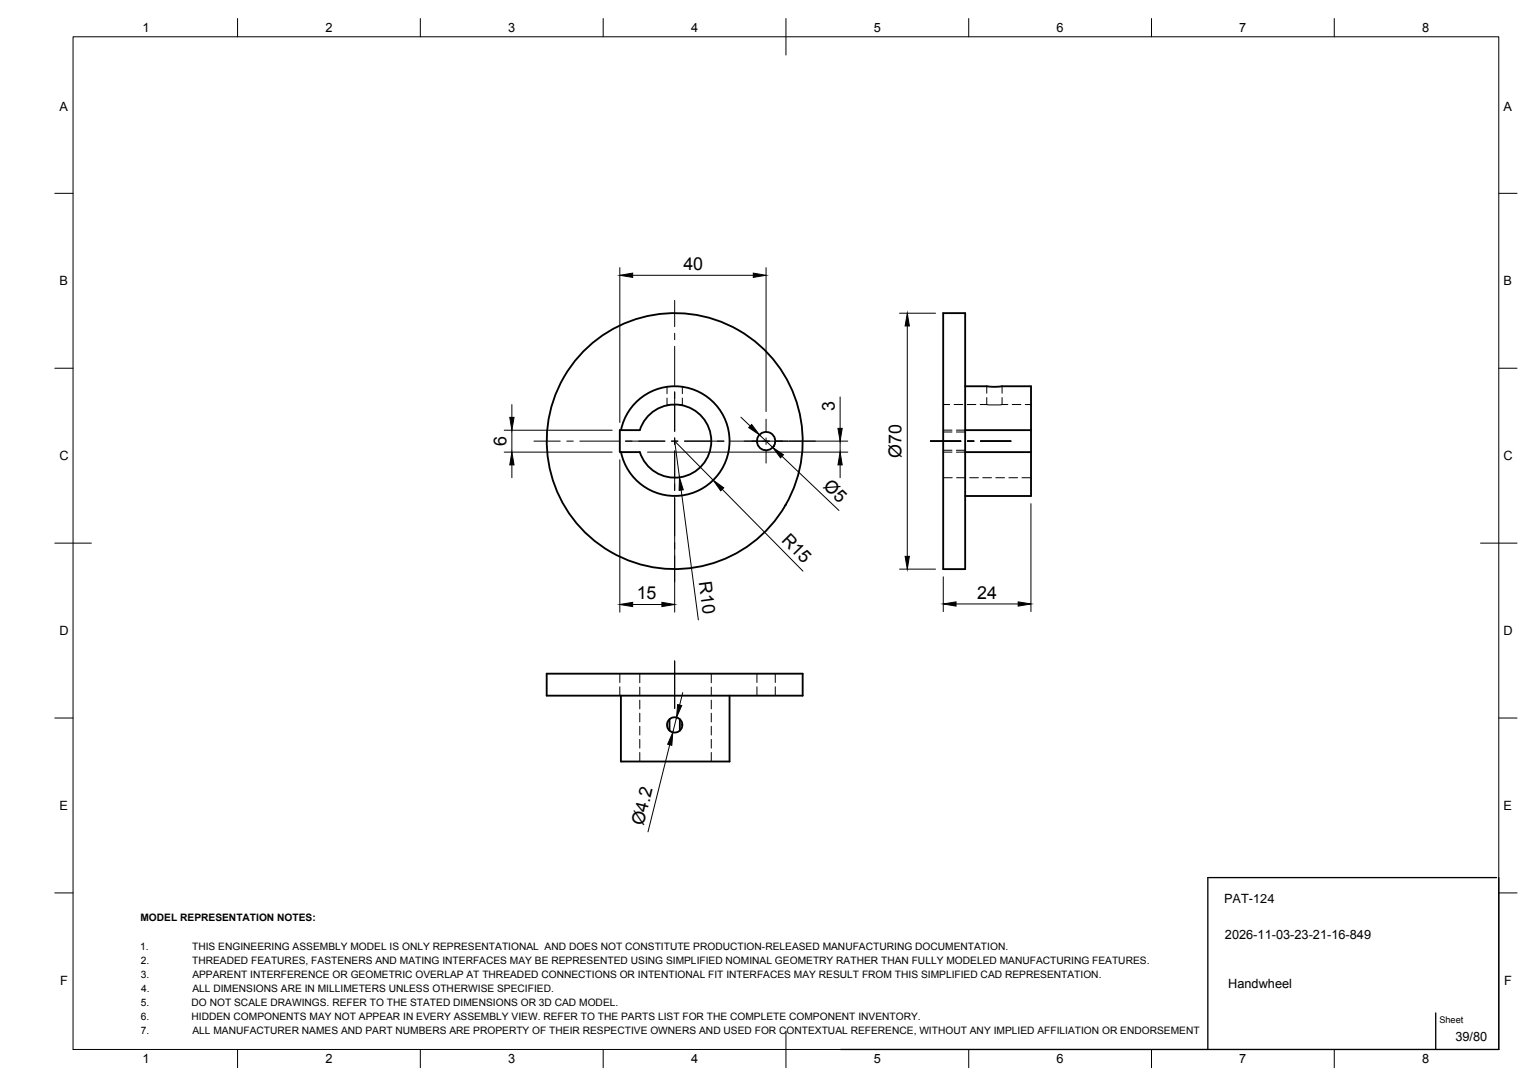
ISO-10303-21;
HEADER;
/* Generated by software containing ST-Developer
 * from STEP Tools, Inc. (www.steptools.com) 
 */

FILE_DESCRIPTION(
/* description */ ('XY cross-slide table'),
/* implementation_level */ '2;1');

FILE_NAME(
/* name */ 'Handwheel.step',
/* time_stamp */ '2026-10-28T03:22:46-07:00',
/* author */ (''),
/* organization */ (''),
/* preprocessor_version */ 'ST-DEVELOPER v20.2',
/* originating_system */ 'Autodesk Translation Framework v15.17.0.0',
/* authorisation */ '');

FILE_SCHEMA (('AUTOMOTIVE_DESIGN { 1 0 10303 214 3 1 1 }'));
ENDSEC;

DATA;
#10=MECHANICAL_DESIGN_GEOMETRIC_PRESENTATION_REPRESENTATION('',(#1720),#62984);
#1032=B_SPLINE_CURVE_WITH_KNOTS('',3,(#47403,#47404,#47405,#47406,#47407,
#47408),.UNSPECIFIED.,.F.,.F.,(4,2,4),(0.803821788694078,0.872950991853625,
0.952307212900975),.UNSPECIFIED.);
#1033=B_SPLINE_CURVE_WITH_KNOTS('',3,(#47411,#47412,#47413,#47414,#47415,
#47416,#47417,#47418,#47419,#47420),.UNSPECIFIED.,.F.,.F.,(4,2,2,2,4),(0.168950313426762,
0.238079516586309,0.317435737633658,0.396791958681008,0.465921161840561),
 .UNSPECIFIED.);
#1034=B_SPLINE_CURVE_WITH_KNOTS('',3,(#47421,#47422,#47423,#47424,#47425,
#47426),.UNSPECIFIED.,.F.,.F.,(4,2,4),(0.952307212900975,1.03166343394832,
1.10079263710787),.UNSPECIFIED.);
#1035=B_SPLINE_CURVE_WITH_KNOTS('',3,(#47430,#47431,#47432,#47433,#47434,
#47435,#47436,#47437,#47438,#47439),.UNSPECIFIED.,.F.,.F.,(4,2,2,2,4),(0.,
0.0792165807733642,0.158433161546728,0.237648697074572,0.316864232602417),
 .UNSPECIFIED.);
#1036=B_SPLINE_CURVE_WITH_KNOTS('',3,(#47440,#47441,#47442,#47443,#47444,
#47445,#47446,#47447,#47448,#47449,#47450,#47451,#47452,#47453,#47454,#47455,
#47456,#47457,#47458,#47459,#47460,#47461,#47462,#47463,#47464,#47465),
 .UNSPECIFIED.,.F.,.F.,(4,2,2,2,2,2,2,2,2,2,2,2,4),(0.316864232602417,0.396079768130261,
0.475295303658105,0.554511884431469,0.633728465204833,0.712945045978197,
0.792161626751562,0.871377162279406,0.95059269780725,1.02980823333509,1.10902376886294,
1.1882403496363,1.26745693040967),.UNSPECIFIED.);
#1539=SHAPE_REPRESENTATION_RELATIONSHIP('SRR','None',#63392,#1622);
#1622=ADVANCED_BREP_SHAPE_REPRESENTATION('',(#1830),#62929);
#1720=STYLED_ITEM('',(#63905),#1830);
#1830=MANIFOLD_SOLID_BREP('Body1',#23017);
#2071=FACE_BOUND('',#4954,.T.);
#2072=FACE_BOUND('',#4955,.T.);
#2073=FACE_BOUND('',#4957,.T.);
#2074=FACE_BOUND('',#4958,.T.);
#2075=FACE_BOUND('',#4961,.T.);
#2076=FACE_BOUND('',#4963,.T.);
#2533=PLANE('',#25052);
#2534=PLANE('',#25056);
#2535=PLANE('',#25057);
#2536=PLANE('',#25058);
#2537=PLANE('',#25059);
#2538=PLANE('',#25060);
#2539=PLANE('',#25063);
#2540=PLANE('',#25071);
#3448=FACE_OUTER_BOUND('',#4946,.T.);
#3449=FACE_OUTER_BOUND('',#4947,.T.);
#3450=FACE_OUTER_BOUND('',#4948,.T.);
#3451=FACE_OUTER_BOUND('',#4949,.T.);
#3452=FACE_OUTER_BOUND('',#4950,.T.);
#3453=FACE_OUTER_BOUND('',#4951,.T.);
#3454=FACE_OUTER_BOUND('',#4952,.T.);
#3455=FACE_OUTER_BOUND('',#4953,.T.);
#3456=FACE_OUTER_BOUND('',#4956,.T.);
#3457=FACE_OUTER_BOUND('',#4959,.T.);
#3458=FACE_OUTER_BOUND('',#4960,.T.);
#3459=FACE_OUTER_BOUND('',#4962,.T.);
#3460=FACE_OUTER_BOUND('',#4964,.T.);
#4946=EDGE_LOOP('',(#17664,#17665,#17666,#17667));
#4947=EDGE_LOOP('',(#17668,#17669));
#4948=EDGE_LOOP('',(#17670,#17671,#17672,#17673,#17674,#17675,#17676,#17677,
#17678));
#4949=EDGE_LOOP('',(#17679,#17680));
#4950=EDGE_LOOP('',(#17681,#17682,#17683,#17684,#17685,#17686));
#4951=EDGE_LOOP('',(#17687,#17688,#17689,#17690));
#4952=EDGE_LOOP('',(#17691,#17692,#17693,#17694,#17695,#17696));
#4953=EDGE_LOOP('',(#17697));
#4954=EDGE_LOOP('',(#17698));
#4955=EDGE_LOOP('',(#17699,#17700,#17701,#17702));
#4956=EDGE_LOOP('',(#17703));
#4957=EDGE_LOOP('',(#17704));
#4958=EDGE_LOOP('',(#17705,#17706,#17707,#17708));
#4959=EDGE_LOOP('',(#17709,#17710,#17711,#17712));
#4960=EDGE_LOOP('',(#17713,#17714,#17715,#17716));
#4961=EDGE_LOOP('',(#17717,#17718,#17719,#17720,#17721));
#4962=EDGE_LOOP('',(#17722,#17723,#17724,#17725));
#4963=EDGE_LOOP('',(#17726,#17727));
#4964=EDGE_LOOP('',(#17728,#17729,#17730,#17731));
#6550=LINE('',#47393,#8037);
#6551=LINE('',#47398,#8038);
#6552=LINE('',#47428,#8039);
#6553=LINE('',#47467,#8040);
#6554=LINE('',#47471,#8041);
#6555=LINE('',#47473,#8042);
#6556=LINE('',#47475,#8043);
#6557=LINE('',#47477,#8044);
#6558=LINE('',#47479,#8045);
#6559=LINE('',#47480,#8046);
#6560=LINE('',#47483,#8047);
#6561=LINE('',#47485,#8048);
#6562=LINE('',#47486,#8049);
#6563=LINE('',#47489,#8050);
#6564=LINE('',#47491,#8051);
#6565=LINE('',#47493,#8052);
#6566=LINE('',#47495,#8053);
#6567=LINE('',#47496,#8054);
#6568=LINE('',#47506,#8055);
#8037=VECTOR('',#29207,0.25);
#8038=VECTOR('',#29212,1.);
#8039=VECTOR('',#29219,0.210000000000001);
#8040=VECTOR('',#29222,1.);
#8041=VECTOR('',#29225,1.);
#8042=VECTOR('',#29226,1.);
#8043=VECTOR('',#29227,1.);
#8044=VECTOR('',#29228,1.);
#8045=VECTOR('',#29229,1.);
#8046=VECTOR('',#29230,1.);
#8047=VECTOR('',#29233,1.);
#8048=VECTOR('',#29234,1.);
#8049=VECTOR('',#29235,1.);
#8050=VECTOR('',#29238,1.);
#8051=VECTOR('',#29239,1.);
#8052=VECTOR('',#29240,1.);
#8053=VECTOR('',#29241,1.);
#8054=VECTOR('',#29242,1.);
#8055=VECTOR('',#29257,3.5);
#9277=CIRCLE('',#25050,0.25);
#9278=CIRCLE('',#25051,0.25);
#9279=CIRCLE('',#25053,0.210000000000001);
#9280=CIRCLE('',#25055,0.210000000000001);
#9281=CIRCLE('',#25061,3.5);
#9282=CIRCLE('',#25062,1.);
#9283=CIRCLE('',#25064,3.5);
#9284=CIRCLE('',#25065,1.5);
#9285=CIRCLE('',#25068,1.);
#9286=CIRCLE('',#25070,1.5);
#10704=VERTEX_POINT('',#47390);
#10705=VERTEX_POINT('',#47392);
#10706=VERTEX_POINT('',#47396);
#10707=VERTEX_POINT('',#47397);
#10708=VERTEX_POINT('',#47401);
#10709=VERTEX_POINT('',#47402);
#10710=VERTEX_POINT('',#47409);
#10711=VERTEX_POINT('',#47427);
#10712=VERTEX_POINT('',#47429);
#10713=VERTEX_POINT('',#47469);
#10714=VERTEX_POINT('',#47470);
#10715=VERTEX_POINT('',#47472);
#10716=VERTEX_POINT('',#47474);
#10717=VERTEX_POINT('',#47476);
#10718=VERTEX_POINT('',#47478);
#10719=VERTEX_POINT('',#47482);
#10720=VERTEX_POINT('',#47484);
#10721=VERTEX_POINT('',#47488);
#10722=VERTEX_POINT('',#47490);
#10723=VERTEX_POINT('',#47492);
#10724=VERTEX_POINT('',#47494);
#10725=VERTEX_POINT('',#47498);
#10726=VERTEX_POINT('',#47502);
#13216=EDGE_CURVE('',#10704,#10704,#9277,.T.);
#13217=EDGE_CURVE('',#10704,#10705,#6550,.T.);
#13218=EDGE_CURVE('',#10705,#10705,#9278,.T.);
#13219=EDGE_CURVE('',#10706,#10707,#6551,.T.);
#13220=EDGE_CURVE('',#10706,#10707,#9279,.T.);
#13221=EDGE_CURVE('',#10708,#10709,#1032,.T.);
#13222=EDGE_CURVE('',#10710,#10708,#9280,.T.);
#13223=EDGE_CURVE('',#10707,#10710,#1033,.T.);
#13224=EDGE_CURVE('',#10709,#10706,#1034,.T.);
#13225=EDGE_CURVE('',#10709,#10711,#6552,.T.);
#13226=EDGE_CURVE('',#10712,#10711,#1035,.T.);
#13227=EDGE_CURVE('',#10711,#10712,#1036,.T.);
#13228=EDGE_CURVE('',#10710,#10708,#6553,.T.);
#13229=EDGE_CURVE('',#10713,#10714,#6554,.T.);
#13230=EDGE_CURVE('',#10715,#10713,#6555,.T.);
#13231=EDGE_CURVE('',#10716,#10715,#6556,.T.);
#13232=EDGE_CURVE('',#10717,#10716,#6557,.T.);
#13233=EDGE_CURVE('',#10718,#10717,#6558,.T.);
#13234=EDGE_CURVE('',#10714,#10718,#6559,.T.);
#13235=EDGE_CURVE('',#10719,#10713,#6560,.T.);
#13236=EDGE_CURVE('',#10720,#10719,#6561,.T.);
#13237=EDGE_CURVE('',#10715,#10720,#6562,.T.);
#13238=EDGE_CURVE('',#10721,#10719,#6563,.T.);
#13239=EDGE_CURVE('',#10722,#10721,#6564,.T.);
#13240=EDGE_CURVE('',#10723,#10722,#6565,.T.);
#13241=EDGE_CURVE('',#10724,#10723,#6566,.T.);
#13242=EDGE_CURVE('',#10720,#10724,#6567,.T.);
#13243=EDGE_CURVE('',#10725,#10725,#9281,.T.);
#13244=EDGE_CURVE('',#10714,#10721,#9282,.T.);
#13245=EDGE_CURVE('',#10726,#10726,#9283,.T.);
#13246=EDGE_CURVE('',#10724,#10716,#9284,.T.);
#13247=EDGE_CURVE('',#10725,#10726,#6568,.T.);
#13248=EDGE_CURVE('',#10718,#10722,#9285,.T.);
#13249=EDGE_CURVE('',#10723,#10717,#9286,.T.);
#17664=ORIENTED_EDGE('',*,*,#13216,.F.);
#17665=ORIENTED_EDGE('',*,*,#13217,.T.);
#17666=ORIENTED_EDGE('',*,*,#13218,.F.);
#17667=ORIENTED_EDGE('',*,*,#13217,.F.);
#17668=ORIENTED_EDGE('',*,*,#13219,.F.);
#17669=ORIENTED_EDGE('',*,*,#13220,.T.);
#17670=ORIENTED_EDGE('',*,*,#13221,.F.);
#17671=ORIENTED_EDGE('',*,*,#13222,.F.);
#17672=ORIENTED_EDGE('',*,*,#13223,.F.);
#17673=ORIENTED_EDGE('',*,*,#13220,.F.);
#17674=ORIENTED_EDGE('',*,*,#13224,.F.);
#17675=ORIENTED_EDGE('',*,*,#13225,.T.);
#17676=ORIENTED_EDGE('',*,*,#13226,.F.);
#17677=ORIENTED_EDGE('',*,*,#13227,.F.);
#17678=ORIENTED_EDGE('',*,*,#13225,.F.);
#17679=ORIENTED_EDGE('',*,*,#13228,.F.);
#17680=ORIENTED_EDGE('',*,*,#13222,.T.);
#17681=ORIENTED_EDGE('',*,*,#13229,.F.);
#17682=ORIENTED_EDGE('',*,*,#13230,.F.);
#17683=ORIENTED_EDGE('',*,*,#13231,.F.);
#17684=ORIENTED_EDGE('',*,*,#13232,.F.);
#17685=ORIENTED_EDGE('',*,*,#13233,.F.);
#17686=ORIENTED_EDGE('',*,*,#13234,.F.);
#17687=ORIENTED_EDGE('',*,*,#13235,.F.);
#17688=ORIENTED_EDGE('',*,*,#13236,.F.);
#17689=ORIENTED_EDGE('',*,*,#13237,.F.);
#17690=ORIENTED_EDGE('',*,*,#13230,.T.);
#17691=ORIENTED_EDGE('',*,*,#13238,.F.);
#17692=ORIENTED_EDGE('',*,*,#13239,.F.);
#17693=ORIENTED_EDGE('',*,*,#13240,.F.);
#17694=ORIENTED_EDGE('',*,*,#13241,.F.);
#17695=ORIENTED_EDGE('',*,*,#13242,.F.);
#17696=ORIENTED_EDGE('',*,*,#13236,.T.);
#17697=ORIENTED_EDGE('',*,*,#13243,.T.);
#17698=ORIENTED_EDGE('',*,*,#13218,.T.);
#17699=ORIENTED_EDGE('',*,*,#13238,.T.);
#17700=ORIENTED_EDGE('',*,*,#13235,.T.);
#17701=ORIENTED_EDGE('',*,*,#13229,.T.);
#17702=ORIENTED_EDGE('',*,*,#13244,.T.);
#17703=ORIENTED_EDGE('',*,*,#13245,.F.);
#17704=ORIENTED_EDGE('',*,*,#13216,.T.);
#17705=ORIENTED_EDGE('',*,*,#13242,.T.);
#17706=ORIENTED_EDGE('',*,*,#13246,.T.);
#17707=ORIENTED_EDGE('',*,*,#13231,.T.);
#17708=ORIENTED_EDGE('',*,*,#13237,.T.);
#17709=ORIENTED_EDGE('',*,*,#13243,.F.);
#17710=ORIENTED_EDGE('',*,*,#13247,.T.);
#17711=ORIENTED_EDGE('',*,*,#13245,.T.);
#17712=ORIENTED_EDGE('',*,*,#13247,.F.);
#17713=ORIENTED_EDGE('',*,*,#13239,.T.);
#17714=ORIENTED_EDGE('',*,*,#13244,.F.);
#17715=ORIENTED_EDGE('',*,*,#13234,.T.);
#17716=ORIENTED_EDGE('',*,*,#13248,.T.);
#17717=ORIENTED_EDGE('',*,*,#13223,.T.);
#17718=ORIENTED_EDGE('',*,*,#13228,.T.);
#17719=ORIENTED_EDGE('',*,*,#13221,.T.);
#17720=ORIENTED_EDGE('',*,*,#13224,.T.);
#17721=ORIENTED_EDGE('',*,*,#13219,.T.);
#17722=ORIENTED_EDGE('',*,*,#13241,.T.);
#17723=ORIENTED_EDGE('',*,*,#13249,.T.);
#17724=ORIENTED_EDGE('',*,*,#13232,.T.);
#17725=ORIENTED_EDGE('',*,*,#13246,.F.);
#17726=ORIENTED_EDGE('',*,*,#13226,.T.);
#17727=ORIENTED_EDGE('',*,*,#13227,.T.);
#17728=ORIENTED_EDGE('',*,*,#13240,.T.);
#17729=ORIENTED_EDGE('',*,*,#13248,.F.);
#17730=ORIENTED_EDGE('',*,*,#13233,.T.);
#17731=ORIENTED_EDGE('',*,*,#13249,.F.);
#21324=CYLINDRICAL_SURFACE('',#25049,0.25);
#21325=CYLINDRICAL_SURFACE('',#25054,0.210000000000001);
#21326=CYLINDRICAL_SURFACE('',#25066,3.5);
#21327=CYLINDRICAL_SURFACE('',#25067,1.);
#21328=CYLINDRICAL_SURFACE('',#25069,1.5);
#22229=ADVANCED_FACE('',(#3448),#21324,.F.);
#22230=ADVANCED_FACE('',(#3449),#2533,.T.);
#22231=ADVANCED_FACE('',(#3450),#21325,.F.);
#22232=ADVANCED_FACE('',(#3451),#2534,.T.);
#22233=ADVANCED_FACE('',(#3452),#2535,.F.);
#22234=ADVANCED_FACE('',(#3453),#2536,.F.);
#22235=ADVANCED_FACE('',(#3454),#2537,.F.);
#22236=ADVANCED_FACE('',(#3455,#2071,#2072),#2538,.T.);
#22237=ADVANCED_FACE('',(#3456,#2073,#2074),#2539,.F.);
#22238=ADVANCED_FACE('',(#3457),#21326,.T.);
#22239=ADVANCED_FACE('',(#3458,#2075),#21327,.F.);
#22240=ADVANCED_FACE('',(#3459,#2076),#21328,.T.);
#22241=ADVANCED_FACE('',(#3460),#2540,.F.);
#23017=CLOSED_SHELL('',(#22229,#22230,#22231,#22232,#22233,#22234,#22235,
#22236,#22237,#22238,#22239,#22240,#22241));
#25048=AXIS2_PLACEMENT_3D('',#47388,#29201,#29202);
#25049=AXIS2_PLACEMENT_3D('',#47389,#29203,#29204);
#25050=AXIS2_PLACEMENT_3D('',#47391,#29205,#29206);
#25051=AXIS2_PLACEMENT_3D('',#47394,#29208,#29209);
#25052=AXIS2_PLACEMENT_3D('',#47395,#29210,#29211);
#25053=AXIS2_PLACEMENT_3D('',#47399,#29213,#29214);
#25054=AXIS2_PLACEMENT_3D('',#47400,#29215,#29216);
#25055=AXIS2_PLACEMENT_3D('',#47410,#29217,#29218);
#25056=AXIS2_PLACEMENT_3D('',#47466,#29220,#29221);
#25057=AXIS2_PLACEMENT_3D('',#47468,#29223,#29224);
#25058=AXIS2_PLACEMENT_3D('',#47481,#29231,#29232);
#25059=AXIS2_PLACEMENT_3D('',#47487,#29236,#29237);
#25060=AXIS2_PLACEMENT_3D('',#47497,#29243,#29244);
#25061=AXIS2_PLACEMENT_3D('',#47499,#29245,#29246);
#25062=AXIS2_PLACEMENT_3D('',#47500,#29247,#29248);
#25063=AXIS2_PLACEMENT_3D('',#47501,#29249,#29250);
#25064=AXIS2_PLACEMENT_3D('',#47503,#29251,#29252);
#25065=AXIS2_PLACEMENT_3D('',#47504,#29253,#29254);
#25066=AXIS2_PLACEMENT_3D('',#47505,#29255,#29256);
#25067=AXIS2_PLACEMENT_3D('',#47507,#29258,#29259);
#25068=AXIS2_PLACEMENT_3D('',#47508,#29260,#29261);
#25069=AXIS2_PLACEMENT_3D('',#47509,#29262,#29263);
#25070=AXIS2_PLACEMENT_3D('',#47510,#29264,#29265);
#25071=AXIS2_PLACEMENT_3D('',#47511,#29266,#29267);
#29201=DIRECTION('axis',(0.,0.,1.));
#29202=DIRECTION('refdir',(1.,0.,0.));
#29203=DIRECTION('center_axis',(1.,0.,0.));
#29204=DIRECTION('ref_axis',(0.,0.,-1.));
#29205=DIRECTION('center_axis',(1.,0.,0.));
#29206=DIRECTION('ref_axis',(0.,0.,-1.));
#29207=DIRECTION('',(1.,0.,0.));
#29208=DIRECTION('center_axis',(-1.,0.,0.));
#29209=DIRECTION('ref_axis',(0.,0.,-1.));
#29210=DIRECTION('center_axis',(0.,1.,0.));
#29211=DIRECTION('ref_axis',(1.,0.,0.));
#29212=DIRECTION('',(1.,0.,0.));
#29213=DIRECTION('center_axis',(0.,1.,0.));
#29214=DIRECTION('ref_axis',(1.,0.,0.));
#29215=DIRECTION('center_axis',(0.,1.,0.));
#29216=DIRECTION('ref_axis',(1.,0.,0.));
#29217=DIRECTION('center_axis',(0.,1.,0.));
#29218=DIRECTION('ref_axis',(1.,0.,0.));
#29219=DIRECTION('',(0.,1.,0.));
#29220=DIRECTION('center_axis',(0.,1.,0.));
#29221=DIRECTION('ref_axis',(1.,0.,0.));
#29222=DIRECTION('',(-1.,0.,0.));
#29223=DIRECTION('center_axis',(0.,-1.,0.));
#29224=DIRECTION('ref_axis',(0.,0.,-1.));
#29225=DIRECTION('',(0.,0.,1.));
#29226=DIRECTION('',(1.,0.,0.));
#29227=DIRECTION('',(0.,0.,-1.));
#29228=DIRECTION('',(1.,0.,0.));
#29229=DIRECTION('',(0.,0.,-1.));
#29230=DIRECTION('',(-1.,0.,0.));
#29231=DIRECTION('center_axis',(0.,0.,-1.));
#29232=DIRECTION('ref_axis',(0.,1.,0.));
#29233=DIRECTION('',(0.,-1.,0.));
#29234=DIRECTION('',(1.,0.,0.));
#29235=DIRECTION('',(0.,1.,0.));
#29236=DIRECTION('center_axis',(0.,1.,0.));
#29237=DIRECTION('ref_axis',(0.,0.,1.));
#29238=DIRECTION('',(0.,0.,-1.));
#29239=DIRECTION('',(1.,0.,0.));
#29240=DIRECTION('',(0.,0.,1.));
#29241=DIRECTION('',(-1.,0.,0.));
#29242=DIRECTION('',(0.,0.,1.));
#29243=DIRECTION('center_axis',(1.,0.,0.));
#29244=DIRECTION('ref_axis',(0.,0.,-1.));
#29245=DIRECTION('center_axis',(1.,0.,0.));
#29246=DIRECTION('ref_axis',(0.,0.,-1.));
#29247=DIRECTION('center_axis',(-1.,0.,0.));
#29248=DIRECTION('ref_axis',(0.,0.,-1.));
#29249=DIRECTION('center_axis',(1.,0.,0.));
#29250=DIRECTION('ref_axis',(0.,0.,-1.));
#29251=DIRECTION('center_axis',(1.,0.,0.));
#29252=DIRECTION('ref_axis',(0.,0.,-1.));
#29253=DIRECTION('center_axis',(1.,0.,0.));
#29254=DIRECTION('ref_axis',(0.,0.,-1.));
#29255=DIRECTION('center_axis',(1.,0.,0.));
#29256=DIRECTION('ref_axis',(0.,0.,-1.));
#29257=DIRECTION('',(-1.,0.,0.));
#29258=DIRECTION('center_axis',(1.,0.,0.));
#29259=DIRECTION('ref_axis',(0.,1.22464679914735E-16,1.));
#29260=DIRECTION('center_axis',(-1.,0.,0.));
#29261=DIRECTION('ref_axis',(0.,0.,-1.));
#29262=DIRECTION('center_axis',(1.,0.,0.));
#29263=DIRECTION('ref_axis',(0.,1.22464679914735E-16,1.));
#29264=DIRECTION('center_axis',(1.,0.,0.));
#29265=DIRECTION('ref_axis',(0.,0.,-1.));
#29266=DIRECTION('center_axis',(1.,0.,0.));
#29267=DIRECTION('ref_axis',(0.,0.,-1.));
#47388=CARTESIAN_POINT('',(0.,0.,0.));
#47389=CARTESIAN_POINT('Origin',(28.7,0.,6.5));
#47390=CARTESIAN_POINT('',(28.8,-3.06161699786838E-17,6.75));
#47391=CARTESIAN_POINT('Origin',(28.8,0.,6.5));
#47392=CARTESIAN_POINT('',(29.4,3.06161699786838E-17,6.75));
#47393=CARTESIAN_POINT('',(28.7,-3.06161699786838E-17,6.75));
#47394=CARTESIAN_POINT('Origin',(29.4,0.,6.5));
#47395=CARTESIAN_POINT('Origin',(28.,0.99,4.));
#47396=CARTESIAN_POINT('',(27.844436508139,0.99,4.14106735979666));
#47397=CARTESIAN_POINT('',(28.155563491861,0.99,4.14106735979666));
#47398=CARTESIAN_POINT('',(27.,0.99,4.14106735979666));
#47399=CARTESIAN_POINT('Origin',(28.,0.99,4.));
#47400=CARTESIAN_POINT('Origin',(28.,0.99,4.));
#47401=CARTESIAN_POINT('',(27.844436508139,0.99,3.85893264020334));
#47402=CARTESIAN_POINT('',(27.79,1.,4.));
#47403=CARTESIAN_POINT('Ctrl Pts',(27.844436508139,0.99,3.85893264020334));
#47404=CARTESIAN_POINT('Ctrl Pts',(27.8287948476368,0.992457849824465,3.87618164330178));
#47405=CARTESIAN_POINT('Ctrl Pts',(27.815375956669,0.994938193049464,3.8970013568903));
#47406=CARTESIAN_POINT('Ctrl Pts',(27.7953025362756,0.998844492372413,3.94538588560165));
#47407=CARTESIAN_POINT('Ctrl Pts',(27.79,1.,3.97354792631755));
#47408=CARTESIAN_POINT('Ctrl Pts',(27.79,1.,4.));
#47409=CARTESIAN_POINT('',(28.155563491861,0.99,3.85893264020334));
#47410=CARTESIAN_POINT('Origin',(28.,0.99,4.));
#47411=CARTESIAN_POINT('Ctrl Pts',(28.155563491861,0.99,4.14106735979666));
#47412=CARTESIAN_POINT('Ctrl Pts',(28.1712051523632,0.992457849824465,4.12381835669823));
#47413=CARTESIAN_POINT('Ctrl Pts',(28.184624043331,0.994938193049464,4.1029986431097));
#47414=CARTESIAN_POINT('Ctrl Pts',(28.2046974637244,0.998844492372413,4.05461411439835));
#47415=CARTESIAN_POINT('Ctrl Pts',(28.21,1.,4.02645207368245));
#47416=CARTESIAN_POINT('Ctrl Pts',(28.21,1.,3.97354792631755));
#47417=CARTESIAN_POINT('Ctrl Pts',(28.2046974637244,0.998844492372413,3.94538588560165));
#47418=CARTESIAN_POINT('Ctrl Pts',(28.184624043331,0.994938193049464,3.8970013568903));
#47419=CARTESIAN_POINT('Ctrl Pts',(28.1712051523632,0.992457849824465,3.87618164330178));
#47420=CARTESIAN_POINT('Ctrl Pts',(28.155563491861,0.99,3.85893264020334));
#47421=CARTESIAN_POINT('Ctrl Pts',(27.79,1.,4.));
#47422=CARTESIAN_POINT('Ctrl Pts',(27.79,1.,4.02645207368245));
#47423=CARTESIAN_POINT('Ctrl Pts',(27.7953025362756,0.998844492372413,4.05461411439835));
#47424=CARTESIAN_POINT('Ctrl Pts',(27.815375956669,0.994938193049464,4.1029986431097));
#47425=CARTESIAN_POINT('Ctrl Pts',(27.8287948476368,0.992457849824465,4.12381835669823));
#47426=CARTESIAN_POINT('Ctrl Pts',(27.844436508139,0.99,4.14106735979666));
#47427=CARTESIAN_POINT('',(27.79,1.5,4.));
#47428=CARTESIAN_POINT('',(27.79,0.99,4.));
#47429=CARTESIAN_POINT('',(28.,1.48522725533839,4.21));
#47430=CARTESIAN_POINT('Ctrl Pts',(28.,1.48522725533839,4.21));
#47431=CARTESIAN_POINT('Ctrl Pts',(27.9735944730755,1.48522725533839,4.21));
#47432=CARTESIAN_POINT('Ctrl Pts',(27.9454529259093,1.48600415954412,4.20471573726959));
#47433=CARTESIAN_POINT('Ctrl Pts',(27.8937237310949,1.48880073282317,4.18327376303633));
#47434=CARTESIAN_POINT('Ctrl Pts',(27.870133075872,1.49077897157582,4.16711792397039));
#47435=CARTESIAN_POINT('Ctrl Pts',(27.832882321789,1.49448481141327,4.12986716988737));
#47436=CARTESIAN_POINT('Ctrl Pts',(27.8167262899986,1.49645455657129,4.10627640830576));
#47437=CARTESIAN_POINT('Ctrl Pts',(27.7952841751738,1.49923165515646,4.0545468514059));
#47438=CARTESIAN_POINT('Ctrl Pts',(27.79,1.5,4.02640517850928));
#47439=CARTESIAN_POINT('Ctrl Pts',(27.79,1.5,4.));
#47440=CARTESIAN_POINT('Ctrl Pts',(27.79,1.5,4.));
#47441=CARTESIAN_POINT('Ctrl Pts',(27.79,1.5,3.97359482149072));
#47442=CARTESIAN_POINT('Ctrl Pts',(27.7952841751738,1.49923165515646,3.9454531485941));
#47443=CARTESIAN_POINT('Ctrl Pts',(27.8167262899986,1.49645455657129,3.89372359169424));
#47444=CARTESIAN_POINT('Ctrl Pts',(27.832882321789,1.49448481141327,3.87013283011263));
#47445=CARTESIAN_POINT('Ctrl Pts',(27.870133075872,1.49077897157582,3.83288207602961));
#47446=CARTESIAN_POINT('Ctrl Pts',(27.8937237310949,1.48880073282317,3.81672623696367));
#47447=CARTESIAN_POINT('Ctrl Pts',(27.9454529259093,1.48600415954412,3.7952842627304));
#47448=CARTESIAN_POINT('Ctrl Pts',(27.9735944730755,1.48522725533839,3.79));
#47449=CARTESIAN_POINT('Ctrl Pts',(28.0264055269245,1.48522725533839,3.79));
#47450=CARTESIAN_POINT('Ctrl Pts',(28.0545470740907,1.48600415954412,3.7952842627304));
#47451=CARTESIAN_POINT('Ctrl Pts',(28.1062762689051,1.48880073282317,3.81672623696367));
#47452=CARTESIAN_POINT('Ctrl Pts',(28.129866924128,1.49077897157582,3.83288207602961));
#47453=CARTESIAN_POINT('Ctrl Pts',(28.167117678211,1.49448481141327,3.87013283011263));
#47454=CARTESIAN_POINT('Ctrl Pts',(28.1832737100014,1.49645455657129,3.89372359169424));
#47455=CARTESIAN_POINT('Ctrl Pts',(28.2047158248262,1.49923165515646,3.9454531485941));
#47456=CARTESIAN_POINT('Ctrl Pts',(28.21,1.5,3.97359482149072));
#47457=CARTESIAN_POINT('Ctrl Pts',(28.21,1.5,4.02640517850928));
#47458=CARTESIAN_POINT('Ctrl Pts',(28.2047158248262,1.49923165515646,4.0545468514059));
#47459=CARTESIAN_POINT('Ctrl Pts',(28.1832737100014,1.49645455657129,4.10627640830576));
#47460=CARTESIAN_POINT('Ctrl Pts',(28.167117678211,1.49448481141327,4.12986716988737));
#47461=CARTESIAN_POINT('Ctrl Pts',(28.129866924128,1.49077897157582,4.16711792397039));
#47462=CARTESIAN_POINT('Ctrl Pts',(28.1062762689051,1.48880073282317,4.18327376303633));
#47463=CARTESIAN_POINT('Ctrl Pts',(28.0545470740907,1.48600415954412,4.2047157372696));
#47464=CARTESIAN_POINT('Ctrl Pts',(28.0264055269245,1.48522725533839,4.21));
#47465=CARTESIAN_POINT('Ctrl Pts',(28.,1.48522725533839,4.21));
#47466=CARTESIAN_POINT('Origin',(28.,0.99,4.));
#47467=CARTESIAN_POINT('',(27.,0.99,3.85893264020334));
#47468=CARTESIAN_POINT('Origin',(26.9,-0.3,4.));
#47469=CARTESIAN_POINT('',(29.4,-0.3,2.5));
#47470=CARTESIAN_POINT('',(29.4,-0.3,3.04606079858305));
#47471=CARTESIAN_POINT('',(29.4,-0.3,4.));
#47472=CARTESIAN_POINT('',(28.8,-0.3,2.5));
#47473=CARTESIAN_POINT('',(26.9,-0.3,2.5));
#47474=CARTESIAN_POINT('',(28.8,-0.3,2.53030615433009));
#47475=CARTESIAN_POINT('',(28.8,-0.3,4.));
#47476=CARTESIAN_POINT('',(27.,-0.3,2.53030615433009));
#47477=CARTESIAN_POINT('',(27.,-0.3,2.53030615433009));
#47478=CARTESIAN_POINT('',(27.,-0.3,3.04606079858305));
#47479=CARTESIAN_POINT('',(27.,-0.3,4.));
#47480=CARTESIAN_POINT('',(27.,-0.3,3.04606079858305));
#47481=CARTESIAN_POINT('Origin',(26.9,-0.3,2.5));
#47482=CARTESIAN_POINT('',(29.4,0.3,2.5));
#47483=CARTESIAN_POINT('',(29.4,-0.15,2.5));
#47484=CARTESIAN_POINT('',(28.8,0.3,2.5));
#47485=CARTESIAN_POINT('',(26.9,0.3,2.5));
#47486=CARTESIAN_POINT('',(28.8,-0.15,2.5));
#47487=CARTESIAN_POINT('Origin',(26.9,0.3,2.5));
#47488=CARTESIAN_POINT('',(29.4,0.3,3.04606079858305));
#47489=CARTESIAN_POINT('',(29.4,0.3,3.25));
#47490=CARTESIAN_POINT('',(27.,0.3,3.04606079858305));
#47491=CARTESIAN_POINT('',(27.,0.3,3.04606079858305));
#47492=CARTESIAN_POINT('',(27.,0.3,2.53030615433009));
#47493=CARTESIAN_POINT('',(27.,0.3,3.25));
#47494=CARTESIAN_POINT('',(28.8,0.3,2.53030615433009));
#47495=CARTESIAN_POINT('',(27.,0.3,2.53030615433009));
#47496=CARTESIAN_POINT('',(28.8,0.3,3.25));
#47497=CARTESIAN_POINT('Origin',(29.4,0.,4.));
#47498=CARTESIAN_POINT('',(29.4,-4.28626379701574E-16,7.5));
#47499=CARTESIAN_POINT('Origin',(29.4,0.,4.));
#47500=CARTESIAN_POINT('Origin',(29.4,0.,4.));
#47501=CARTESIAN_POINT('Origin',(28.8,0.,4.));
#47502=CARTESIAN_POINT('',(28.8,-4.28626379701574E-16,7.5));
#47503=CARTESIAN_POINT('Origin',(28.8,0.,4.));
#47504=CARTESIAN_POINT('Origin',(28.8,0.,4.));
#47505=CARTESIAN_POINT('Origin',(28.8,0.,4.));
#47506=CARTESIAN_POINT('',(28.8,-4.28626379701574E-16,7.5));
#47507=CARTESIAN_POINT('Origin',(27.,0.,4.));
#47508=CARTESIAN_POINT('Origin',(27.,0.,4.));
#47509=CARTESIAN_POINT('Origin',(27.,0.,4.));
#47510=CARTESIAN_POINT('Origin',(27.,0.,4.));
#47511=CARTESIAN_POINT('Origin',(27.,0.,4.));
#62830=UNCERTAINTY_MEASURE_WITH_UNIT(LENGTH_MEASURE(0.001),#62985,
'DISTANCE_ACCURACY_VALUE',
'Maximum model space distance between geometric entities at asserted c
onnectivities');
#62885=UNCERTAINTY_MEASURE_WITH_UNIT(LENGTH_MEASURE(0.001),#62985,
'DISTANCE_ACCURACY_VALUE',
'Maximum model space distance between geometric entities at asserted c
onnectivities');
#62929=(
GEOMETRIC_REPRESENTATION_CONTEXT(3)
GLOBAL_UNCERTAINTY_ASSIGNED_CONTEXT((#62830))
GLOBAL_UNIT_ASSIGNED_CONTEXT((#62985,#62987,#62988))
REPRESENTATION_CONTEXT('','3D')
);
#62984=(
GEOMETRIC_REPRESENTATION_CONTEXT(3)
GLOBAL_UNCERTAINTY_ASSIGNED_CONTEXT((#62885))
GLOBAL_UNIT_ASSIGNED_CONTEXT((#62985,#62987,#62988))
REPRESENTATION_CONTEXT('','3D')
);
#62985=(
LENGTH_UNIT()
NAMED_UNIT(*)
SI_UNIT(.CENTI.,.METRE.)
);
#62987=(
NAMED_UNIT(*)
PLANE_ANGLE_UNIT()
SI_UNIT($,.RADIAN.)
);
#62988=(
NAMED_UNIT(*)
SI_UNIT($,.STERADIAN.)
SOLID_ANGLE_UNIT()
);
#63032=SHAPE_DEFINITION_REPRESENTATION(#63163,#63392);
#63163=PRODUCT_DEFINITION_SHAPE('',$,#63491);
#63392=SHAPE_REPRESENTATION('',(#25048),#62929);
#63447=PRODUCT_DEFINITION_CONTEXT('part definition',#63743,'design');
#63491=PRODUCT_DEFINITION('Handwheel','Handwheel',#63589,#63447);
#63589=PRODUCT_DEFINITION_FORMATION('',$,#63788);
#63743=APPLICATION_CONTEXT(
'Core Data for Automotive Mechanical Design Process');
#63744=PRODUCT_CONTEXT('part definition',#63743,'mechanical');
#63788=PRODUCT('Handwheel','Handwheel','Handwheel',(#63744));
#63899=COLOUR_RGB('Sky Blue',0.24,0.69,0.87);
#63900=FILL_AREA_STYLE_COLOUR('',#63899);
#63901=FILL_AREA_STYLE('',(#63900));
#63902=SURFACE_STYLE_FILL_AREA(#63901);
#63903=SURFACE_SIDE_STYLE('',(#63902));
#63904=SURFACE_STYLE_USAGE(.BOTH.,#63903);
#63905=PRESENTATION_STYLE_ASSIGNMENT((#63904));
ENDSEC;
END-ISO-10303-21;
